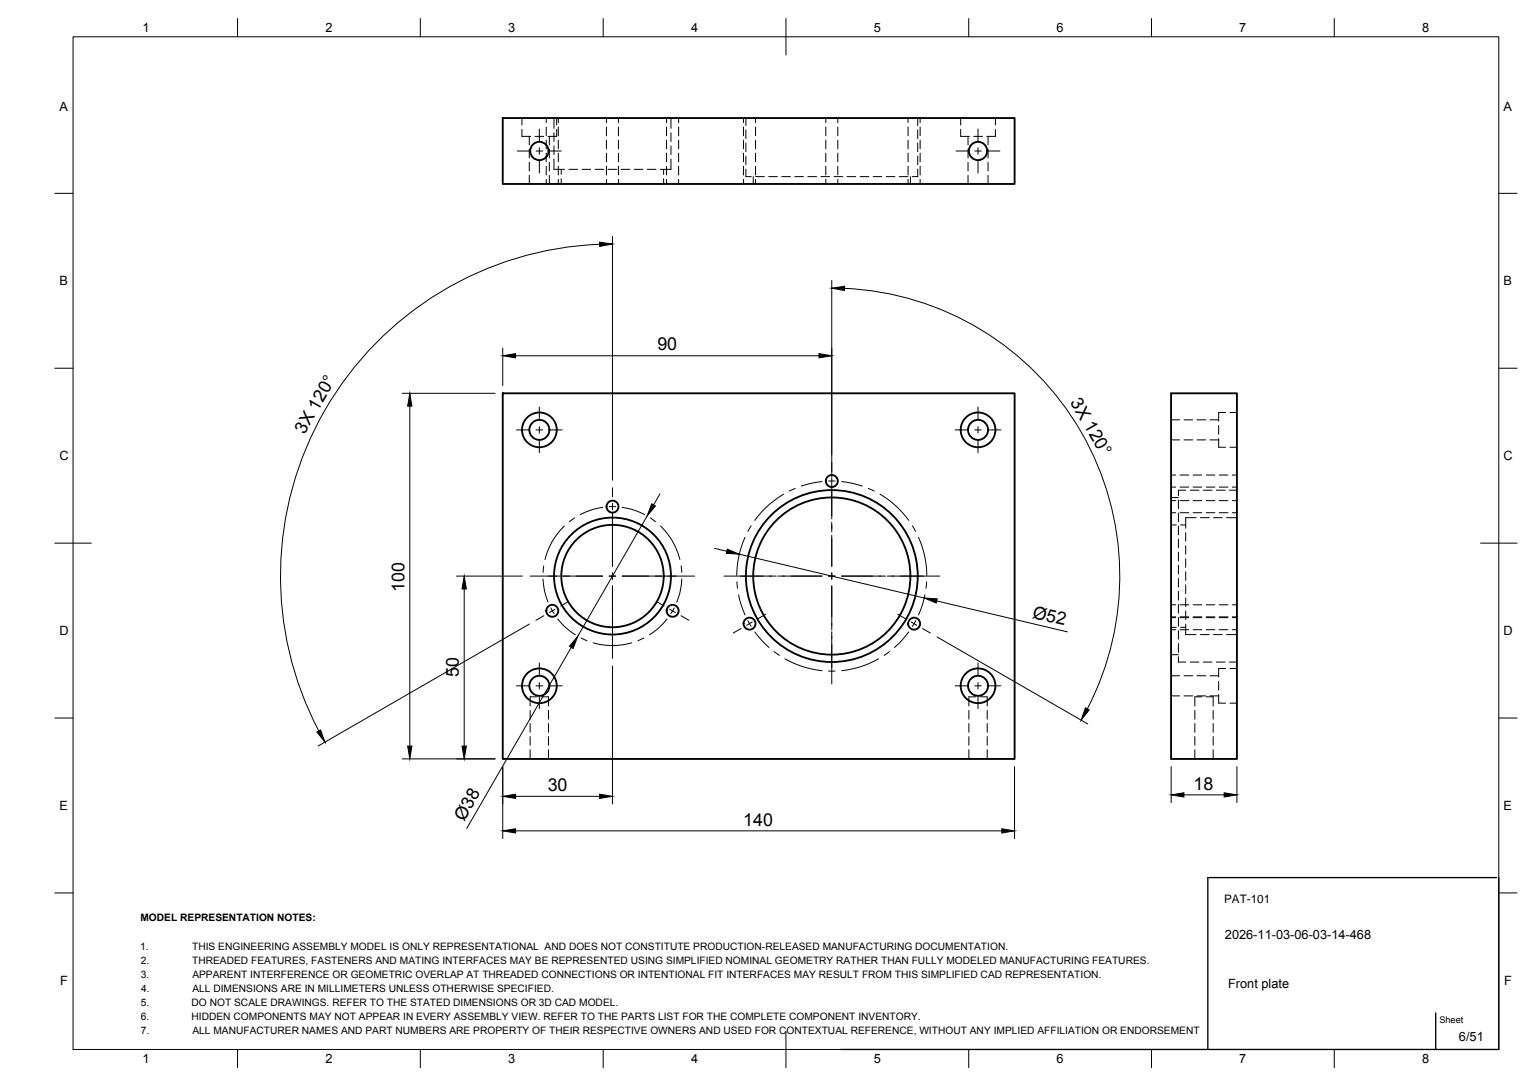
ISO-10303-21;
HEADER;
/* Generated by software containing ST-Developer
 * from STEP Tools, Inc. (www.steptools.com) 
 */

FILE_DESCRIPTION(
/* description */ ('Spur gear reduction stage 2-1 on bearing plates'),
/* implementation_level */ '2;1');

FILE_NAME(
/* name */ 'Front plate.step',
/* time_stamp */ '2026-10-28T03:22:07-07:00',
/* author */ (''),
/* organization */ (''),
/* preprocessor_version */ 'ST-DEVELOPER v20.2',
/* originating_system */ 'Autodesk Translation Framework v15.17.0.0',
/* authorisation */ '');

FILE_SCHEMA (('AUTOMOTIVE_DESIGN { 1 0 10303 214 3 1 1 }'));
ENDSEC;

DATA;
#10=MECHANICAL_DESIGN_GEOMETRIC_PRESENTATION_REPRESENTATION('',(#948),#53909);
#862=SHAPE_REPRESENTATION_RELATIONSHIP('SRR','None',#54089,#905);
#905=ADVANCED_BREP_SHAPE_REPRESENTATION('',(#1006),#53863);
#948=STYLED_ITEM('',(#54411),#1006);
#1006=MANIFOLD_SOLID_BREP('Body1',#11272);
#1068=FACE_BOUND('',#2177,.T.);
#1069=FACE_BOUND('',#2180,.T.);
#1070=FACE_BOUND('',#2183,.T.);
#1071=FACE_BOUND('',#2186,.T.);
#1072=FACE_BOUND('',#2197,.T.);
#1073=FACE_BOUND('',#2201,.T.);
#1074=FACE_BOUND('',#2204,.T.);
#1075=FACE_BOUND('',#2205,.T.);
#1076=FACE_BOUND('',#2206,.T.);
#1077=FACE_BOUND('',#2207,.T.);
#1078=FACE_BOUND('',#2208,.T.);
#1079=FACE_BOUND('',#2209,.T.);
#1080=FACE_BOUND('',#2210,.T.);
#1081=FACE_BOUND('',#2211,.T.);
#1082=FACE_BOUND('',#2212,.T.);
#1083=FACE_BOUND('',#2213,.T.);
#1084=FACE_BOUND('',#2214,.T.);
#1085=FACE_BOUND('',#2215,.T.);
#1086=FACE_BOUND('',#2218,.T.);
#1087=FACE_BOUND('',#2219,.T.);
#1088=FACE_BOUND('',#2220,.T.);
#1089=FACE_BOUND('',#2221,.T.);
#1090=FACE_BOUND('',#2222,.T.);
#1091=FACE_BOUND('',#2223,.T.);
#1092=FACE_BOUND('',#2224,.T.);
#1093=FACE_BOUND('',#2225,.T.);
#1094=FACE_BOUND('',#2226,.T.);
#1095=FACE_BOUND('',#2227,.T.);
#1096=FACE_BOUND('',#2228,.T.);
#1097=FACE_BOUND('',#2229,.T.);
#1098=FACE_BOUND('',#2233,.T.);
#1099=FACE_BOUND('',#2234,.T.);
#1244=PLANE('',#11849);
#1245=PLANE('',#11854);
#1246=PLANE('',#11859);
#1247=PLANE('',#11864);
#1248=PLANE('',#11877);
#1249=PLANE('',#11881);
#1250=PLANE('',#11885);
#1251=PLANE('',#11892);
#1252=PLANE('',#11896);
#1253=PLANE('',#11897);
#1254=PLANE('',#11898);
#1255=PLANE('',#11899);
#1256=PLANE('',#11900);
#1257=PLANE('',#11901);
#1513=FACE_OUTER_BOUND('',#2169,.T.);
#1514=FACE_OUTER_BOUND('',#2170,.T.);
#1515=FACE_OUTER_BOUND('',#2171,.T.);
#1516=FACE_OUTER_BOUND('',#2172,.T.);
#1517=FACE_OUTER_BOUND('',#2173,.T.);
#1518=FACE_OUTER_BOUND('',#2174,.T.);
#1519=FACE_OUTER_BOUND('',#2175,.T.);
#1520=FACE_OUTER_BOUND('',#2176,.T.);
#1521=FACE_OUTER_BOUND('',#2178,.T.);
#1522=FACE_OUTER_BOUND('',#2179,.T.);
#1523=FACE_OUTER_BOUND('',#2181,.T.);
#1524=FACE_OUTER_BOUND('',#2182,.T.);
#1525=FACE_OUTER_BOUND('',#2184,.T.);
#1526=FACE_OUTER_BOUND('',#2185,.T.);
#1527=FACE_OUTER_BOUND('',#2187,.T.);
#1528=FACE_OUTER_BOUND('',#2188,.T.);
#1529=FACE_OUTER_BOUND('',#2189,.T.);
#1530=FACE_OUTER_BOUND('',#2190,.T.);
#1531=FACE_OUTER_BOUND('',#2191,.T.);
#1532=FACE_OUTER_BOUND('',#2192,.T.);
#1533=FACE_OUTER_BOUND('',#2193,.T.);
#1534=FACE_OUTER_BOUND('',#2194,.T.);
#1535=FACE_OUTER_BOUND('',#2195,.T.);
#1536=FACE_OUTER_BOUND('',#2196,.T.);
#1537=FACE_OUTER_BOUND('',#2198,.T.);
#1538=FACE_OUTER_BOUND('',#2199,.T.);
#1539=FACE_OUTER_BOUND('',#2200,.T.);
#1540=FACE_OUTER_BOUND('',#2202,.T.);
#1541=FACE_OUTER_BOUND('',#2203,.T.);
#1542=FACE_OUTER_BOUND('',#2216,.T.);
#1543=FACE_OUTER_BOUND('',#2217,.T.);
#1544=FACE_OUTER_BOUND('',#2230,.T.);
#1545=FACE_OUTER_BOUND('',#2231,.T.);
#1546=FACE_OUTER_BOUND('',#2232,.T.);
#2169=EDGE_LOOP('',(#7400,#7401,#7402,#7403));
#2170=EDGE_LOOP('',(#7404,#7405,#7406,#7407));
#2171=EDGE_LOOP('',(#7408,#7409,#7410,#7411));
#2172=EDGE_LOOP('',(#7412,#7413,#7414,#7415));
#2173=EDGE_LOOP('',(#7416,#7417,#7418,#7419));
#2174=EDGE_LOOP('',(#7420,#7421,#7422,#7423));
#2175=EDGE_LOOP('',(#7424,#7425,#7426,#7427));
#2176=EDGE_LOOP('',(#7428));
#2177=EDGE_LOOP('',(#7429));
#2178=EDGE_LOOP('',(#7430,#7431,#7432,#7433));
#2179=EDGE_LOOP('',(#7434));
#2180=EDGE_LOOP('',(#7435));
#2181=EDGE_LOOP('',(#7436,#7437,#7438,#7439));
#2182=EDGE_LOOP('',(#7440));
#2183=EDGE_LOOP('',(#7441));
#2184=EDGE_LOOP('',(#7442,#7443,#7444,#7445));
#2185=EDGE_LOOP('',(#7446));
#2186=EDGE_LOOP('',(#7447));
#2187=EDGE_LOOP('',(#7448,#7449,#7450,#7451));
#2188=EDGE_LOOP('',(#7452,#7453,#7454,#7455));
#2189=EDGE_LOOP('',(#7456,#7457,#7458,#7459));
#2190=EDGE_LOOP('',(#7460,#7461,#7462,#7463));
#2191=EDGE_LOOP('',(#7464,#7465,#7466,#7467));
#2192=EDGE_LOOP('',(#7468));
#2193=EDGE_LOOP('',(#7469,#7470,#7471,#7472));
#2194=EDGE_LOOP('',(#7473));
#2195=EDGE_LOOP('',(#7474,#7475,#7476,#7477));
#2196=EDGE_LOOP('',(#7478));
#2197=EDGE_LOOP('',(#7479));
#2198=EDGE_LOOP('',(#7480,#7481,#7482,#7483));
#2199=EDGE_LOOP('',(#7484,#7485,#7486,#7487));
#2200=EDGE_LOOP('',(#7488));
#2201=EDGE_LOOP('',(#7489));
#2202=EDGE_LOOP('',(#7490,#7491,#7492,#7493));
#2203=EDGE_LOOP('',(#7494,#7495,#7496,#7497));
#2204=EDGE_LOOP('',(#7498));
#2205=EDGE_LOOP('',(#7499));
#2206=EDGE_LOOP('',(#7500));
#2207=EDGE_LOOP('',(#7501));
#2208=EDGE_LOOP('',(#7502));
#2209=EDGE_LOOP('',(#7503));
#2210=EDGE_LOOP('',(#7504));
#2211=EDGE_LOOP('',(#7505));
#2212=EDGE_LOOP('',(#7506));
#2213=EDGE_LOOP('',(#7507));
#2214=EDGE_LOOP('',(#7508));
#2215=EDGE_LOOP('',(#7509));
#2216=EDGE_LOOP('',(#7510,#7511,#7512,#7513));
#2217=EDGE_LOOP('',(#7514,#7515,#7516,#7517));
#2218=EDGE_LOOP('',(#7518));
#2219=EDGE_LOOP('',(#7519));
#2220=EDGE_LOOP('',(#7520));
#2221=EDGE_LOOP('',(#7521));
#2222=EDGE_LOOP('',(#7522));
#2223=EDGE_LOOP('',(#7523));
#2224=EDGE_LOOP('',(#7524));
#2225=EDGE_LOOP('',(#7525));
#2226=EDGE_LOOP('',(#7526));
#2227=EDGE_LOOP('',(#7527));
#2228=EDGE_LOOP('',(#7528));
#2229=EDGE_LOOP('',(#7529));
#2230=EDGE_LOOP('',(#7530,#7531,#7532,#7533));
#2231=EDGE_LOOP('',(#7534,#7535,#7536,#7537));
#2232=EDGE_LOOP('',(#7538,#7539,#7540,#7541));
#2233=EDGE_LOOP('',(#7542));
#2234=EDGE_LOOP('',(#7543));
#2993=LINE('',#16033,#3634);
#2994=LINE('',#16039,#3635);
#2995=LINE('',#16045,#3636);
#2996=LINE('',#16051,#3637);
#2997=LINE('',#16057,#3638);
#2998=LINE('',#16063,#3639);
#2999=LINE('',#16069,#3640);
#3000=LINE('',#16078,#3641);
#3001=LINE('',#16087,#3642);
#3002=LINE('',#16096,#3643);
#3003=LINE('',#16103,#3644);
#3004=LINE('',#16107,#3645);
#3005=LINE('',#16111,#3646);
#3006=LINE('',#16115,#3647);
#3007=LINE('',#16121,#3648);
#3008=LINE('',#16128,#3649);
#3009=LINE('',#16135,#3650);
#3010=LINE('',#16142,#3651);
#3011=LINE('',#16148,#3652);
#3012=LINE('',#16155,#3653);
#3013=LINE('',#16160,#3654);
#3014=LINE('',#16162,#3655);
#3015=LINE('',#16164,#3656);
#3016=LINE('',#16165,#3657);
#3017=LINE('',#16168,#3658);
#3018=LINE('',#16170,#3659);
#3019=LINE('',#16171,#3660);
#3020=LINE('',#16174,#3661);
#3021=LINE('',#16176,#3662);
#3022=LINE('',#16177,#3663);
#3023=LINE('',#16179,#3664);
#3024=LINE('',#16180,#3665);
#3634=VECTOR('',#13046,0.165);
#3635=VECTOR('',#13053,0.165);
#3636=VECTOR('',#13060,0.164999999999999);
#3637=VECTOR('',#13067,0.165);
#3638=VECTOR('',#13074,0.165);
#3639=VECTOR('',#13081,0.165);
#3640=VECTOR('',#13088,0.475);
#3641=VECTOR('',#13099,0.475);
#3642=VECTOR('',#13110,0.475);
#3643=VECTOR('',#13121,0.475);
#3644=VECTOR('',#13130,0.275);
#3645=VECTOR('',#13135,0.275);
#3646=VECTOR('',#13140,0.275);
#3647=VECTOR('',#13145,0.275);
#3648=VECTOR('',#13152,0.25);
#3649=VECTOR('',#13161,0.25);
#3650=VECTOR('',#13170,2.35);
#3651=VECTOR('',#13179,2.15);
#3652=VECTOR('',#13186,1.6);
#3653=VECTOR('',#13195,1.4);
#3654=VECTOR('',#13200,1.);
#3655=VECTOR('',#13201,1.);
#3656=VECTOR('',#13202,1.);
#3657=VECTOR('',#13203,1.);
#3658=VECTOR('',#13206,1.);
#3659=VECTOR('',#13207,1.);
#3660=VECTOR('',#13208,1.);
#3661=VECTOR('',#13211,1.);
#3662=VECTOR('',#13212,1.);
#3663=VECTOR('',#13213,1.);
#3664=VECTOR('',#13216,1.);
#3665=VECTOR('',#13217,1.);
#4267=CIRCLE('',#11829,0.165);
#4268=CIRCLE('',#11830,0.165);
#4269=CIRCLE('',#11832,0.165);
#4270=CIRCLE('',#11833,0.165);
#4271=CIRCLE('',#11835,0.164999999999999);
#4272=CIRCLE('',#11836,0.164999999999999);
#4273=CIRCLE('',#11838,0.165);
#4274=CIRCLE('',#11839,0.165);
#4275=CIRCLE('',#11841,0.165);
#4276=CIRCLE('',#11842,0.165);
#4277=CIRCLE('',#11844,0.165);
#4278=CIRCLE('',#11845,0.165);
#4279=CIRCLE('',#11847,0.475);
#4280=CIRCLE('',#11848,0.475);
#4281=CIRCLE('',#11850,0.275);
#4282=CIRCLE('',#11852,0.475);
#4283=CIRCLE('',#11853,0.475);
#4284=CIRCLE('',#11855,0.275);
#4285=CIRCLE('',#11857,0.475);
#4286=CIRCLE('',#11858,0.475);
#4287=CIRCLE('',#11860,0.275);
#4288=CIRCLE('',#11862,0.475);
#4289=CIRCLE('',#11863,0.475);
#4290=CIRCLE('',#11865,0.275);
#4291=CIRCLE('',#11867,0.275);
#4292=CIRCLE('',#11869,0.275);
#4293=CIRCLE('',#11871,0.275);
#4294=CIRCLE('',#11873,0.275);
#4295=CIRCLE('',#11875,0.25);
#4296=CIRCLE('',#11876,0.25);
#4297=CIRCLE('',#11879,0.25);
#4298=CIRCLE('',#11880,0.25);
#4299=CIRCLE('',#11883,2.35);
#4300=CIRCLE('',#11884,2.35);
#4301=CIRCLE('',#11886,2.15);
#4302=CIRCLE('',#11888,2.15);
#4303=CIRCLE('',#11890,1.6);
#4304=CIRCLE('',#11891,1.6);
#4305=CIRCLE('',#11893,1.4);
#4306=CIRCLE('',#11895,1.4);
#4800=VERTEX_POINT('',#16030);
#4801=VERTEX_POINT('',#16032);
#4802=VERTEX_POINT('',#16036);
#4803=VERTEX_POINT('',#16038);
#4804=VERTEX_POINT('',#16042);
#4805=VERTEX_POINT('',#16044);
#4806=VERTEX_POINT('',#16048);
#4807=VERTEX_POINT('',#16050);
#4808=VERTEX_POINT('',#16054);
#4809=VERTEX_POINT('',#16056);
#4810=VERTEX_POINT('',#16060);
#4811=VERTEX_POINT('',#16062);
#4812=VERTEX_POINT('',#16066);
#4813=VERTEX_POINT('',#16068);
#4814=VERTEX_POINT('',#16072);
#4815=VERTEX_POINT('',#16075);
#4816=VERTEX_POINT('',#16077);
#4817=VERTEX_POINT('',#16081);
#4818=VERTEX_POINT('',#16084);
#4819=VERTEX_POINT('',#16086);
#4820=VERTEX_POINT('',#16090);
#4821=VERTEX_POINT('',#16093);
#4822=VERTEX_POINT('',#16095);
#4823=VERTEX_POINT('',#16099);
#4824=VERTEX_POINT('',#16102);
#4825=VERTEX_POINT('',#16106);
#4826=VERTEX_POINT('',#16110);
#4827=VERTEX_POINT('',#16114);
#4828=VERTEX_POINT('',#16118);
#4829=VERTEX_POINT('',#16120);
#4830=VERTEX_POINT('',#16125);
#4831=VERTEX_POINT('',#16127);
#4832=VERTEX_POINT('',#16132);
#4833=VERTEX_POINT('',#16134);
#4834=VERTEX_POINT('',#16138);
#4835=VERTEX_POINT('',#16141);
#4836=VERTEX_POINT('',#16145);
#4837=VERTEX_POINT('',#16147);
#4838=VERTEX_POINT('',#16151);
#4839=VERTEX_POINT('',#16154);
#4840=VERTEX_POINT('',#16158);
#4841=VERTEX_POINT('',#16159);
#4842=VERTEX_POINT('',#16161);
#4843=VERTEX_POINT('',#16163);
#4844=VERTEX_POINT('',#16167);
#4845=VERTEX_POINT('',#16169);
#4846=VERTEX_POINT('',#16173);
#4847=VERTEX_POINT('',#16175);
#5842=EDGE_CURVE('',#4800,#4800,#4267,.T.);
#5843=EDGE_CURVE('',#4800,#4801,#2993,.T.);
#5844=EDGE_CURVE('',#4801,#4801,#4268,.T.);
#5845=EDGE_CURVE('',#4802,#4802,#4269,.T.);
#5846=EDGE_CURVE('',#4802,#4803,#2994,.T.);
#5847=EDGE_CURVE('',#4803,#4803,#4270,.T.);
#5848=EDGE_CURVE('',#4804,#4804,#4271,.T.);
#5849=EDGE_CURVE('',#4804,#4805,#2995,.T.);
#5850=EDGE_CURVE('',#4805,#4805,#4272,.T.);
#5851=EDGE_CURVE('',#4806,#4806,#4273,.T.);
#5852=EDGE_CURVE('',#4806,#4807,#2996,.T.);
#5853=EDGE_CURVE('',#4807,#4807,#4274,.T.);
#5854=EDGE_CURVE('',#4808,#4808,#4275,.T.);
#5855=EDGE_CURVE('',#4808,#4809,#2997,.T.);
#5856=EDGE_CURVE('',#4809,#4809,#4276,.T.);
#5857=EDGE_CURVE('',#4810,#4810,#4277,.T.);
#5858=EDGE_CURVE('',#4810,#4811,#2998,.T.);
#5859=EDGE_CURVE('',#4811,#4811,#4278,.T.);
#5860=EDGE_CURVE('',#4812,#4812,#4279,.T.);
#5861=EDGE_CURVE('',#4812,#4813,#2999,.T.);
#5862=EDGE_CURVE('',#4813,#4813,#4280,.T.);
#5863=EDGE_CURVE('',#4814,#4814,#4281,.T.);
#5864=EDGE_CURVE('',#4815,#4815,#4282,.T.);
#5865=EDGE_CURVE('',#4815,#4816,#3000,.T.);
#5866=EDGE_CURVE('',#4816,#4816,#4283,.T.);
#5867=EDGE_CURVE('',#4817,#4817,#4284,.T.);
#5868=EDGE_CURVE('',#4818,#4818,#4285,.T.);
#5869=EDGE_CURVE('',#4818,#4819,#3001,.T.);
#5870=EDGE_CURVE('',#4819,#4819,#4286,.T.);
#5871=EDGE_CURVE('',#4820,#4820,#4287,.T.);
#5872=EDGE_CURVE('',#4821,#4821,#4288,.T.);
#5873=EDGE_CURVE('',#4821,#4822,#3002,.T.);
#5874=EDGE_CURVE('',#4822,#4822,#4289,.T.);
#5875=EDGE_CURVE('',#4823,#4823,#4290,.T.);
#5876=EDGE_CURVE('',#4814,#4824,#3003,.T.);
#5877=EDGE_CURVE('',#4824,#4824,#4291,.T.);
#5878=EDGE_CURVE('',#4817,#4825,#3004,.T.);
#5879=EDGE_CURVE('',#4825,#4825,#4292,.T.);
#5880=EDGE_CURVE('',#4820,#4826,#3005,.T.);
#5881=EDGE_CURVE('',#4826,#4826,#4293,.T.);
#5882=EDGE_CURVE('',#4823,#4827,#3006,.T.);
#5883=EDGE_CURVE('',#4827,#4827,#4294,.T.);
#5884=EDGE_CURVE('',#4828,#4828,#4295,.T.);
#5885=EDGE_CURVE('',#4828,#4829,#3007,.T.);
#5886=EDGE_CURVE('',#4829,#4829,#4296,.T.);
#5887=EDGE_CURVE('',#4830,#4830,#4297,.T.);
#5888=EDGE_CURVE('',#4830,#4831,#3008,.T.);
#5889=EDGE_CURVE('',#4831,#4831,#4298,.T.);
#5890=EDGE_CURVE('',#4832,#4832,#4299,.T.);
#5891=EDGE_CURVE('',#4832,#4833,#3009,.T.);
#5892=EDGE_CURVE('',#4833,#4833,#4300,.T.);
#5893=EDGE_CURVE('',#4834,#4834,#4301,.T.);
#5894=EDGE_CURVE('',#4834,#4835,#3010,.T.);
#5895=EDGE_CURVE('',#4835,#4835,#4302,.T.);
#5896=EDGE_CURVE('',#4836,#4836,#4303,.T.);
#5897=EDGE_CURVE('',#4836,#4837,#3011,.T.);
#5898=EDGE_CURVE('',#4837,#4837,#4304,.T.);
#5899=EDGE_CURVE('',#4838,#4838,#4305,.T.);
#5900=EDGE_CURVE('',#4838,#4839,#3012,.T.);
#5901=EDGE_CURVE('',#4839,#4839,#4306,.T.);
#5902=EDGE_CURVE('',#4840,#4841,#3013,.T.);
#5903=EDGE_CURVE('',#4841,#4842,#3014,.T.);
#5904=EDGE_CURVE('',#4843,#4842,#3015,.T.);
#5905=EDGE_CURVE('',#4840,#4843,#3016,.T.);
#5906=EDGE_CURVE('',#4844,#4840,#3017,.T.);
#5907=EDGE_CURVE('',#4845,#4843,#3018,.T.);
#5908=EDGE_CURVE('',#4844,#4845,#3019,.T.);
#5909=EDGE_CURVE('',#4846,#4844,#3020,.T.);
#5910=EDGE_CURVE('',#4847,#4845,#3021,.T.);
#5911=EDGE_CURVE('',#4846,#4847,#3022,.T.);
#5912=EDGE_CURVE('',#4841,#4846,#3023,.T.);
#5913=EDGE_CURVE('',#4842,#4847,#3024,.T.);
#7400=ORIENTED_EDGE('',*,*,#5842,.F.);
#7401=ORIENTED_EDGE('',*,*,#5843,.T.);
#7402=ORIENTED_EDGE('',*,*,#5844,.F.);
#7403=ORIENTED_EDGE('',*,*,#5843,.F.);
#7404=ORIENTED_EDGE('',*,*,#5845,.F.);
#7405=ORIENTED_EDGE('',*,*,#5846,.T.);
#7406=ORIENTED_EDGE('',*,*,#5847,.F.);
#7407=ORIENTED_EDGE('',*,*,#5846,.F.);
#7408=ORIENTED_EDGE('',*,*,#5848,.F.);
#7409=ORIENTED_EDGE('',*,*,#5849,.T.);
#7410=ORIENTED_EDGE('',*,*,#5850,.F.);
#7411=ORIENTED_EDGE('',*,*,#5849,.F.);
#7412=ORIENTED_EDGE('',*,*,#5851,.F.);
#7413=ORIENTED_EDGE('',*,*,#5852,.T.);
#7414=ORIENTED_EDGE('',*,*,#5853,.F.);
#7415=ORIENTED_EDGE('',*,*,#5852,.F.);
#7416=ORIENTED_EDGE('',*,*,#5854,.F.);
#7417=ORIENTED_EDGE('',*,*,#5855,.T.);
#7418=ORIENTED_EDGE('',*,*,#5856,.F.);
#7419=ORIENTED_EDGE('',*,*,#5855,.F.);
#7420=ORIENTED_EDGE('',*,*,#5857,.F.);
#7421=ORIENTED_EDGE('',*,*,#5858,.T.);
#7422=ORIENTED_EDGE('',*,*,#5859,.F.);
#7423=ORIENTED_EDGE('',*,*,#5858,.F.);
#7424=ORIENTED_EDGE('',*,*,#5860,.F.);
#7425=ORIENTED_EDGE('',*,*,#5861,.T.);
#7426=ORIENTED_EDGE('',*,*,#5862,.T.);
#7427=ORIENTED_EDGE('',*,*,#5861,.F.);
#7428=ORIENTED_EDGE('',*,*,#5862,.F.);
#7429=ORIENTED_EDGE('',*,*,#5863,.F.);
#7430=ORIENTED_EDGE('',*,*,#5864,.F.);
#7431=ORIENTED_EDGE('',*,*,#5865,.T.);
#7432=ORIENTED_EDGE('',*,*,#5866,.T.);
#7433=ORIENTED_EDGE('',*,*,#5865,.F.);
#7434=ORIENTED_EDGE('',*,*,#5866,.F.);
#7435=ORIENTED_EDGE('',*,*,#5867,.F.);
#7436=ORIENTED_EDGE('',*,*,#5868,.F.);
#7437=ORIENTED_EDGE('',*,*,#5869,.T.);
#7438=ORIENTED_EDGE('',*,*,#5870,.T.);
#7439=ORIENTED_EDGE('',*,*,#5869,.F.);
#7440=ORIENTED_EDGE('',*,*,#5870,.F.);
#7441=ORIENTED_EDGE('',*,*,#5871,.F.);
#7442=ORIENTED_EDGE('',*,*,#5872,.F.);
#7443=ORIENTED_EDGE('',*,*,#5873,.T.);
#7444=ORIENTED_EDGE('',*,*,#5874,.T.);
#7445=ORIENTED_EDGE('',*,*,#5873,.F.);
#7446=ORIENTED_EDGE('',*,*,#5874,.F.);
#7447=ORIENTED_EDGE('',*,*,#5875,.F.);
#7448=ORIENTED_EDGE('',*,*,#5863,.T.);
#7449=ORIENTED_EDGE('',*,*,#5876,.T.);
#7450=ORIENTED_EDGE('',*,*,#5877,.F.);
#7451=ORIENTED_EDGE('',*,*,#5876,.F.);
#7452=ORIENTED_EDGE('',*,*,#5867,.T.);
#7453=ORIENTED_EDGE('',*,*,#5878,.T.);
#7454=ORIENTED_EDGE('',*,*,#5879,.F.);
#7455=ORIENTED_EDGE('',*,*,#5878,.F.);
#7456=ORIENTED_EDGE('',*,*,#5871,.T.);
#7457=ORIENTED_EDGE('',*,*,#5880,.T.);
#7458=ORIENTED_EDGE('',*,*,#5881,.F.);
#7459=ORIENTED_EDGE('',*,*,#5880,.F.);
#7460=ORIENTED_EDGE('',*,*,#5875,.T.);
#7461=ORIENTED_EDGE('',*,*,#5882,.T.);
#7462=ORIENTED_EDGE('',*,*,#5883,.F.);
#7463=ORIENTED_EDGE('',*,*,#5882,.F.);
#7464=ORIENTED_EDGE('',*,*,#5884,.F.);
#7465=ORIENTED_EDGE('',*,*,#5885,.T.);
#7466=ORIENTED_EDGE('',*,*,#5886,.T.);
#7467=ORIENTED_EDGE('',*,*,#5885,.F.);
#7468=ORIENTED_EDGE('',*,*,#5886,.F.);
#7469=ORIENTED_EDGE('',*,*,#5887,.F.);
#7470=ORIENTED_EDGE('',*,*,#5888,.T.);
#7471=ORIENTED_EDGE('',*,*,#5889,.T.);
#7472=ORIENTED_EDGE('',*,*,#5888,.F.);
#7473=ORIENTED_EDGE('',*,*,#5889,.F.);
#7474=ORIENTED_EDGE('',*,*,#5890,.F.);
#7475=ORIENTED_EDGE('',*,*,#5891,.T.);
#7476=ORIENTED_EDGE('',*,*,#5892,.T.);
#7477=ORIENTED_EDGE('',*,*,#5891,.F.);
#7478=ORIENTED_EDGE('',*,*,#5892,.F.);
#7479=ORIENTED_EDGE('',*,*,#5893,.F.);
#7480=ORIENTED_EDGE('',*,*,#5893,.T.);
#7481=ORIENTED_EDGE('',*,*,#5894,.T.);
#7482=ORIENTED_EDGE('',*,*,#5895,.F.);
#7483=ORIENTED_EDGE('',*,*,#5894,.F.);
#7484=ORIENTED_EDGE('',*,*,#5896,.F.);
#7485=ORIENTED_EDGE('',*,*,#5897,.T.);
#7486=ORIENTED_EDGE('',*,*,#5898,.T.);
#7487=ORIENTED_EDGE('',*,*,#5897,.F.);
#7488=ORIENTED_EDGE('',*,*,#5898,.F.);
#7489=ORIENTED_EDGE('',*,*,#5899,.F.);
#7490=ORIENTED_EDGE('',*,*,#5899,.T.);
#7491=ORIENTED_EDGE('',*,*,#5900,.T.);
#7492=ORIENTED_EDGE('',*,*,#5901,.F.);
#7493=ORIENTED_EDGE('',*,*,#5900,.F.);
#7494=ORIENTED_EDGE('',*,*,#5902,.T.);
#7495=ORIENTED_EDGE('',*,*,#5903,.T.);
#7496=ORIENTED_EDGE('',*,*,#5904,.F.);
#7497=ORIENTED_EDGE('',*,*,#5905,.F.);
#7498=ORIENTED_EDGE('',*,*,#5853,.T.);
#7499=ORIENTED_EDGE('',*,*,#5856,.T.);
#7500=ORIENTED_EDGE('',*,*,#5859,.T.);
#7501=ORIENTED_EDGE('',*,*,#5901,.T.);
#7502=ORIENTED_EDGE('',*,*,#5895,.T.);
#7503=ORIENTED_EDGE('',*,*,#5883,.T.);
#7504=ORIENTED_EDGE('',*,*,#5881,.T.);
#7505=ORIENTED_EDGE('',*,*,#5879,.T.);
#7506=ORIENTED_EDGE('',*,*,#5877,.T.);
#7507=ORIENTED_EDGE('',*,*,#5850,.T.);
#7508=ORIENTED_EDGE('',*,*,#5847,.T.);
#7509=ORIENTED_EDGE('',*,*,#5844,.T.);
#7510=ORIENTED_EDGE('',*,*,#5906,.T.);
#7511=ORIENTED_EDGE('',*,*,#5905,.T.);
#7512=ORIENTED_EDGE('',*,*,#5907,.F.);
#7513=ORIENTED_EDGE('',*,*,#5908,.F.);
#7514=ORIENTED_EDGE('',*,*,#5909,.T.);
#7515=ORIENTED_EDGE('',*,*,#5908,.T.);
#7516=ORIENTED_EDGE('',*,*,#5910,.F.);
#7517=ORIENTED_EDGE('',*,*,#5911,.F.);
#7518=ORIENTED_EDGE('',*,*,#5851,.T.);
#7519=ORIENTED_EDGE('',*,*,#5854,.T.);
#7520=ORIENTED_EDGE('',*,*,#5857,.T.);
#7521=ORIENTED_EDGE('',*,*,#5890,.T.);
#7522=ORIENTED_EDGE('',*,*,#5896,.T.);
#7523=ORIENTED_EDGE('',*,*,#5872,.T.);
#7524=ORIENTED_EDGE('',*,*,#5868,.T.);
#7525=ORIENTED_EDGE('',*,*,#5864,.T.);
#7526=ORIENTED_EDGE('',*,*,#5860,.T.);
#7527=ORIENTED_EDGE('',*,*,#5848,.T.);
#7528=ORIENTED_EDGE('',*,*,#5845,.T.);
#7529=ORIENTED_EDGE('',*,*,#5842,.T.);
#7530=ORIENTED_EDGE('',*,*,#5912,.T.);
#7531=ORIENTED_EDGE('',*,*,#5911,.T.);
#7532=ORIENTED_EDGE('',*,*,#5913,.F.);
#7533=ORIENTED_EDGE('',*,*,#5903,.F.);
#7534=ORIENTED_EDGE('',*,*,#5913,.T.);
#7535=ORIENTED_EDGE('',*,*,#5910,.T.);
#7536=ORIENTED_EDGE('',*,*,#5907,.T.);
#7537=ORIENTED_EDGE('',*,*,#5904,.T.);
#7538=ORIENTED_EDGE('',*,*,#5912,.F.);
#7539=ORIENTED_EDGE('',*,*,#5902,.F.);
#7540=ORIENTED_EDGE('',*,*,#5906,.F.);
#7541=ORIENTED_EDGE('',*,*,#5909,.F.);
#7542=ORIENTED_EDGE('',*,*,#5884,.T.);
#7543=ORIENTED_EDGE('',*,*,#5887,.T.);
#10424=CYLINDRICAL_SURFACE('',#11828,0.165);
#10425=CYLINDRICAL_SURFACE('',#11831,0.165);
#10426=CYLINDRICAL_SURFACE('',#11834,0.164999999999999);
#10427=CYLINDRICAL_SURFACE('',#11837,0.165);
#10428=CYLINDRICAL_SURFACE('',#11840,0.165);
#10429=CYLINDRICAL_SURFACE('',#11843,0.165);
#10430=CYLINDRICAL_SURFACE('',#11846,0.475);
#10431=CYLINDRICAL_SURFACE('',#11851,0.475);
#10432=CYLINDRICAL_SURFACE('',#11856,0.475);
#10433=CYLINDRICAL_SURFACE('',#11861,0.475);
#10434=CYLINDRICAL_SURFACE('',#11866,0.275);
#10435=CYLINDRICAL_SURFACE('',#11868,0.275);
#10436=CYLINDRICAL_SURFACE('',#11870,0.275);
#10437=CYLINDRICAL_SURFACE('',#11872,0.275);
#10438=CYLINDRICAL_SURFACE('',#11874,0.25);
#10439=CYLINDRICAL_SURFACE('',#11878,0.25);
#10440=CYLINDRICAL_SURFACE('',#11882,2.35);
#10441=CYLINDRICAL_SURFACE('',#11887,2.15);
#10442=CYLINDRICAL_SURFACE('',#11889,1.6);
#10443=CYLINDRICAL_SURFACE('',#11894,1.4);
#10633=ADVANCED_FACE('',(#1513),#10424,.F.);
#10634=ADVANCED_FACE('',(#1514),#10425,.F.);
#10635=ADVANCED_FACE('',(#1515),#10426,.F.);
#10636=ADVANCED_FACE('',(#1516),#10427,.F.);
#10637=ADVANCED_FACE('',(#1517),#10428,.F.);
#10638=ADVANCED_FACE('',(#1518),#10429,.F.);
#10639=ADVANCED_FACE('',(#1519),#10430,.F.);
#10640=ADVANCED_FACE('',(#1520,#1068),#1244,.F.);
#10641=ADVANCED_FACE('',(#1521),#10431,.F.);
#10642=ADVANCED_FACE('',(#1522,#1069),#1245,.F.);
#10643=ADVANCED_FACE('',(#1523),#10432,.F.);
#10644=ADVANCED_FACE('',(#1524,#1070),#1246,.F.);
#10645=ADVANCED_FACE('',(#1525),#10433,.F.);
#10646=ADVANCED_FACE('',(#1526,#1071),#1247,.F.);
#10647=ADVANCED_FACE('',(#1527),#10434,.F.);
#10648=ADVANCED_FACE('',(#1528),#10435,.F.);
#10649=ADVANCED_FACE('',(#1529),#10436,.F.);
#10650=ADVANCED_FACE('',(#1530),#10437,.F.);
#10651=ADVANCED_FACE('',(#1531),#10438,.F.);
#10652=ADVANCED_FACE('',(#1532),#1248,.F.);
#10653=ADVANCED_FACE('',(#1533),#10439,.F.);
#10654=ADVANCED_FACE('',(#1534),#1249,.F.);
#10655=ADVANCED_FACE('',(#1535),#10440,.F.);
#10656=ADVANCED_FACE('',(#1536,#1072),#1250,.F.);
#10657=ADVANCED_FACE('',(#1537),#10441,.F.);
#10658=ADVANCED_FACE('',(#1538),#10442,.F.);
#10659=ADVANCED_FACE('',(#1539,#1073),#1251,.F.);
#10660=ADVANCED_FACE('',(#1540),#10443,.F.);
#10661=ADVANCED_FACE('',(#1541,#1074,#1075,#1076,#1077,#1078,#1079,#1080,
#1081,#1082,#1083,#1084,#1085),#1252,.T.);
#10662=ADVANCED_FACE('',(#1542),#1253,.T.);
#10663=ADVANCED_FACE('',(#1543,#1086,#1087,#1088,#1089,#1090,#1091,#1092,
#1093,#1094,#1095,#1096,#1097),#1254,.T.);
#10664=ADVANCED_FACE('',(#1544),#1255,.T.);
#10665=ADVANCED_FACE('',(#1545),#1256,.T.);
#10666=ADVANCED_FACE('',(#1546,#1098,#1099),#1257,.F.);
#11272=CLOSED_SHELL('',(#10633,#10634,#10635,#10636,#10637,#10638,#10639,
#10640,#10641,#10642,#10643,#10644,#10645,#10646,#10647,#10648,#10649,#10650,
#10651,#10652,#10653,#10654,#10655,#10656,#10657,#10658,#10659,#10660,#10661,
#10662,#10663,#10664,#10665,#10666));
#11827=AXIS2_PLACEMENT_3D('',#16028,#13040,#13041);
#11828=AXIS2_PLACEMENT_3D('',#16029,#13042,#13043);
#11829=AXIS2_PLACEMENT_3D('',#16031,#13044,#13045);
#11830=AXIS2_PLACEMENT_3D('',#16034,#13047,#13048);
#11831=AXIS2_PLACEMENT_3D('',#16035,#13049,#13050);
#11832=AXIS2_PLACEMENT_3D('',#16037,#13051,#13052);
#11833=AXIS2_PLACEMENT_3D('',#16040,#13054,#13055);
#11834=AXIS2_PLACEMENT_3D('',#16041,#13056,#13057);
#11835=AXIS2_PLACEMENT_3D('',#16043,#13058,#13059);
#11836=AXIS2_PLACEMENT_3D('',#16046,#13061,#13062);
#11837=AXIS2_PLACEMENT_3D('',#16047,#13063,#13064);
#11838=AXIS2_PLACEMENT_3D('',#16049,#13065,#13066);
#11839=AXIS2_PLACEMENT_3D('',#16052,#13068,#13069);
#11840=AXIS2_PLACEMENT_3D('',#16053,#13070,#13071);
#11841=AXIS2_PLACEMENT_3D('',#16055,#13072,#13073);
#11842=AXIS2_PLACEMENT_3D('',#16058,#13075,#13076);
#11843=AXIS2_PLACEMENT_3D('',#16059,#13077,#13078);
#11844=AXIS2_PLACEMENT_3D('',#16061,#13079,#13080);
#11845=AXIS2_PLACEMENT_3D('',#16064,#13082,#13083);
#11846=AXIS2_PLACEMENT_3D('',#16065,#13084,#13085);
#11847=AXIS2_PLACEMENT_3D('',#16067,#13086,#13087);
#11848=AXIS2_PLACEMENT_3D('',#16070,#13089,#13090);
#11849=AXIS2_PLACEMENT_3D('',#16071,#13091,#13092);
#11850=AXIS2_PLACEMENT_3D('',#16073,#13093,#13094);
#11851=AXIS2_PLACEMENT_3D('',#16074,#13095,#13096);
#11852=AXIS2_PLACEMENT_3D('',#16076,#13097,#13098);
#11853=AXIS2_PLACEMENT_3D('',#16079,#13100,#13101);
#11854=AXIS2_PLACEMENT_3D('',#16080,#13102,#13103);
#11855=AXIS2_PLACEMENT_3D('',#16082,#13104,#13105);
#11856=AXIS2_PLACEMENT_3D('',#16083,#13106,#13107);
#11857=AXIS2_PLACEMENT_3D('',#16085,#13108,#13109);
#11858=AXIS2_PLACEMENT_3D('',#16088,#13111,#13112);
#11859=AXIS2_PLACEMENT_3D('',#16089,#13113,#13114);
#11860=AXIS2_PLACEMENT_3D('',#16091,#13115,#13116);
#11861=AXIS2_PLACEMENT_3D('',#16092,#13117,#13118);
#11862=AXIS2_PLACEMENT_3D('',#16094,#13119,#13120);
#11863=AXIS2_PLACEMENT_3D('',#16097,#13122,#13123);
#11864=AXIS2_PLACEMENT_3D('',#16098,#13124,#13125);
#11865=AXIS2_PLACEMENT_3D('',#16100,#13126,#13127);
#11866=AXIS2_PLACEMENT_3D('',#16101,#13128,#13129);
#11867=AXIS2_PLACEMENT_3D('',#16104,#13131,#13132);
#11868=AXIS2_PLACEMENT_3D('',#16105,#13133,#13134);
#11869=AXIS2_PLACEMENT_3D('',#16108,#13136,#13137);
#11870=AXIS2_PLACEMENT_3D('',#16109,#13138,#13139);
#11871=AXIS2_PLACEMENT_3D('',#16112,#13141,#13142);
#11872=AXIS2_PLACEMENT_3D('',#16113,#13143,#13144);
#11873=AXIS2_PLACEMENT_3D('',#16116,#13146,#13147);
#11874=AXIS2_PLACEMENT_3D('',#16117,#13148,#13149);
#11875=AXIS2_PLACEMENT_3D('',#16119,#13150,#13151);
#11876=AXIS2_PLACEMENT_3D('',#16122,#13153,#13154);
#11877=AXIS2_PLACEMENT_3D('',#16123,#13155,#13156);
#11878=AXIS2_PLACEMENT_3D('',#16124,#13157,#13158);
#11879=AXIS2_PLACEMENT_3D('',#16126,#13159,#13160);
#11880=AXIS2_PLACEMENT_3D('',#16129,#13162,#13163);
#11881=AXIS2_PLACEMENT_3D('',#16130,#13164,#13165);
#11882=AXIS2_PLACEMENT_3D('',#16131,#13166,#13167);
#11883=AXIS2_PLACEMENT_3D('',#16133,#13168,#13169);
#11884=AXIS2_PLACEMENT_3D('',#16136,#13171,#13172);
#11885=AXIS2_PLACEMENT_3D('',#16137,#13173,#13174);
#11886=AXIS2_PLACEMENT_3D('',#16139,#13175,#13176);
#11887=AXIS2_PLACEMENT_3D('',#16140,#13177,#13178);
#11888=AXIS2_PLACEMENT_3D('',#16143,#13180,#13181);
#11889=AXIS2_PLACEMENT_3D('',#16144,#13182,#13183);
#11890=AXIS2_PLACEMENT_3D('',#16146,#13184,#13185);
#11891=AXIS2_PLACEMENT_3D('',#16149,#13187,#13188);
#11892=AXIS2_PLACEMENT_3D('',#16150,#13189,#13190);
#11893=AXIS2_PLACEMENT_3D('',#16152,#13191,#13192);
#11894=AXIS2_PLACEMENT_3D('',#16153,#13193,#13194);
#11895=AXIS2_PLACEMENT_3D('',#16156,#13196,#13197);
#11896=AXIS2_PLACEMENT_3D('',#16157,#13198,#13199);
#11897=AXIS2_PLACEMENT_3D('',#16166,#13204,#13205);
#11898=AXIS2_PLACEMENT_3D('',#16172,#13209,#13210);
#11899=AXIS2_PLACEMENT_3D('',#16178,#13214,#13215);
#11900=AXIS2_PLACEMENT_3D('',#16181,#13218,#13219);
#11901=AXIS2_PLACEMENT_3D('',#16182,#13220,#13221);
#13040=DIRECTION('axis',(0.,0.,1.));
#13041=DIRECTION('refdir',(1.,0.,0.));
#13042=DIRECTION('center_axis',(0.,1.,0.));
#13043=DIRECTION('ref_axis',(1.,0.,0.));
#13044=DIRECTION('center_axis',(0.,1.,0.));
#13045=DIRECTION('ref_axis',(1.,0.,0.));
#13046=DIRECTION('',(0.,1.,0.));
#13047=DIRECTION('center_axis',(0.,-1.,0.));
#13048=DIRECTION('ref_axis',(1.,0.,0.));
#13049=DIRECTION('center_axis',(0.,1.,0.));
#13050=DIRECTION('ref_axis',(1.,0.,0.));
#13051=DIRECTION('center_axis',(0.,1.,0.));
#13052=DIRECTION('ref_axis',(1.,0.,0.));
#13053=DIRECTION('',(0.,1.,0.));
#13054=DIRECTION('center_axis',(0.,-1.,0.));
#13055=DIRECTION('ref_axis',(1.,0.,0.));
#13056=DIRECTION('center_axis',(0.,1.,0.));
#13057=DIRECTION('ref_axis',(1.,0.,0.));
#13058=DIRECTION('center_axis',(0.,1.,0.));
#13059=DIRECTION('ref_axis',(1.,0.,0.));
#13060=DIRECTION('',(0.,1.,0.));
#13061=DIRECTION('center_axis',(0.,-1.,0.));
#13062=DIRECTION('ref_axis',(1.,0.,0.));
#13063=DIRECTION('center_axis',(0.,1.,0.));
#13064=DIRECTION('ref_axis',(1.,0.,0.));
#13065=DIRECTION('center_axis',(0.,1.,0.));
#13066=DIRECTION('ref_axis',(1.,0.,0.));
#13067=DIRECTION('',(0.,1.,0.));
#13068=DIRECTION('center_axis',(0.,-1.,0.));
#13069=DIRECTION('ref_axis',(1.,0.,0.));
#13070=DIRECTION('center_axis',(0.,1.,0.));
#13071=DIRECTION('ref_axis',(1.,0.,0.));
#13072=DIRECTION('center_axis',(0.,1.,0.));
#13073=DIRECTION('ref_axis',(1.,0.,0.));
#13074=DIRECTION('',(0.,1.,0.));
#13075=DIRECTION('center_axis',(0.,-1.,0.));
#13076=DIRECTION('ref_axis',(1.,0.,0.));
#13077=DIRECTION('center_axis',(0.,1.,0.));
#13078=DIRECTION('ref_axis',(1.,0.,0.));
#13079=DIRECTION('center_axis',(0.,1.,0.));
#13080=DIRECTION('ref_axis',(1.,0.,0.));
#13081=DIRECTION('',(0.,1.,0.));
#13082=DIRECTION('center_axis',(0.,-1.,0.));
#13083=DIRECTION('ref_axis',(1.,0.,0.));
#13084=DIRECTION('center_axis',(0.,1.,0.));
#13085=DIRECTION('ref_axis',(1.,0.,0.));
#13086=DIRECTION('center_axis',(0.,1.,0.));
#13087=DIRECTION('ref_axis',(1.,0.,0.));
#13088=DIRECTION('',(0.,1.,0.));
#13089=DIRECTION('center_axis',(0.,1.,0.));
#13090=DIRECTION('ref_axis',(1.,0.,0.));
#13091=DIRECTION('center_axis',(0.,1.,0.));
#13092=DIRECTION('ref_axis',(1.,0.,0.));
#13093=DIRECTION('center_axis',(0.,-1.,0.));
#13094=DIRECTION('ref_axis',(1.,0.,0.));
#13095=DIRECTION('center_axis',(0.,1.,0.));
#13096=DIRECTION('ref_axis',(1.,0.,0.));
#13097=DIRECTION('center_axis',(0.,1.,0.));
#13098=DIRECTION('ref_axis',(1.,0.,0.));
#13099=DIRECTION('',(0.,1.,0.));
#13100=DIRECTION('center_axis',(0.,1.,0.));
#13101=DIRECTION('ref_axis',(1.,0.,0.));
#13102=DIRECTION('center_axis',(0.,1.,0.));
#13103=DIRECTION('ref_axis',(1.,0.,0.));
#13104=DIRECTION('center_axis',(0.,-1.,0.));
#13105=DIRECTION('ref_axis',(1.,0.,0.));
#13106=DIRECTION('center_axis',(0.,1.,0.));
#13107=DIRECTION('ref_axis',(1.,0.,0.));
#13108=DIRECTION('center_axis',(0.,1.,0.));
#13109=DIRECTION('ref_axis',(1.,0.,0.));
#13110=DIRECTION('',(0.,1.,0.));
#13111=DIRECTION('center_axis',(0.,1.,0.));
#13112=DIRECTION('ref_axis',(1.,0.,0.));
#13113=DIRECTION('center_axis',(0.,1.,0.));
#13114=DIRECTION('ref_axis',(1.,0.,0.));
#13115=DIRECTION('center_axis',(0.,-1.,0.));
#13116=DIRECTION('ref_axis',(1.,0.,0.));
#13117=DIRECTION('center_axis',(0.,1.,0.));
#13118=DIRECTION('ref_axis',(1.,0.,0.));
#13119=DIRECTION('center_axis',(0.,1.,0.));
#13120=DIRECTION('ref_axis',(1.,0.,0.));
#13121=DIRECTION('',(0.,1.,0.));
#13122=DIRECTION('center_axis',(0.,1.,0.));
#13123=DIRECTION('ref_axis',(1.,0.,0.));
#13124=DIRECTION('center_axis',(0.,1.,0.));
#13125=DIRECTION('ref_axis',(1.,0.,0.));
#13126=DIRECTION('center_axis',(0.,-1.,0.));
#13127=DIRECTION('ref_axis',(1.,0.,0.));
#13128=DIRECTION('center_axis',(0.,1.,0.));
#13129=DIRECTION('ref_axis',(1.,0.,0.));
#13130=DIRECTION('',(0.,1.,0.));
#13131=DIRECTION('center_axis',(0.,-1.,0.));
#13132=DIRECTION('ref_axis',(1.,0.,0.));
#13133=DIRECTION('center_axis',(0.,1.,0.));
#13134=DIRECTION('ref_axis',(1.,0.,0.));
#13135=DIRECTION('',(0.,1.,0.));
#13136=DIRECTION('center_axis',(0.,-1.,0.));
#13137=DIRECTION('ref_axis',(1.,0.,0.));
#13138=DIRECTION('center_axis',(0.,1.,0.));
#13139=DIRECTION('ref_axis',(1.,0.,0.));
#13140=DIRECTION('',(0.,1.,0.));
#13141=DIRECTION('center_axis',(0.,-1.,0.));
#13142=DIRECTION('ref_axis',(1.,0.,0.));
#13143=DIRECTION('center_axis',(0.,1.,0.));
#13144=DIRECTION('ref_axis',(1.,0.,0.));
#13145=DIRECTION('',(0.,1.,0.));
#13146=DIRECTION('center_axis',(0.,-1.,0.));
#13147=DIRECTION('ref_axis',(1.,0.,0.));
#13148=DIRECTION('center_axis',(0.,0.,1.));
#13149=DIRECTION('ref_axis',(1.,0.,0.));
#13150=DIRECTION('center_axis',(0.,0.,1.));
#13151=DIRECTION('ref_axis',(1.,0.,0.));
#13152=DIRECTION('',(0.,0.,1.));
#13153=DIRECTION('center_axis',(0.,0.,1.));
#13154=DIRECTION('ref_axis',(1.,0.,0.));
#13155=DIRECTION('center_axis',(0.,0.,1.));
#13156=DIRECTION('ref_axis',(1.,0.,0.));
#13157=DIRECTION('center_axis',(0.,0.,1.));
#13158=DIRECTION('ref_axis',(1.,0.,0.));
#13159=DIRECTION('center_axis',(0.,0.,1.));
#13160=DIRECTION('ref_axis',(1.,0.,0.));
#13161=DIRECTION('',(0.,0.,1.));
#13162=DIRECTION('center_axis',(0.,0.,1.));
#13163=DIRECTION('ref_axis',(1.,0.,0.));
#13164=DIRECTION('center_axis',(0.,0.,1.));
#13165=DIRECTION('ref_axis',(1.,0.,0.));
#13166=DIRECTION('center_axis',(0.,1.,0.));
#13167=DIRECTION('ref_axis',(1.,0.,0.));
#13168=DIRECTION('center_axis',(0.,1.,0.));
#13169=DIRECTION('ref_axis',(1.,0.,0.));
#13170=DIRECTION('',(0.,1.,0.));
#13171=DIRECTION('center_axis',(0.,1.,0.));
#13172=DIRECTION('ref_axis',(1.,0.,0.));
#13173=DIRECTION('center_axis',(0.,1.,0.));
#13174=DIRECTION('ref_axis',(1.,0.,0.));
#13175=DIRECTION('center_axis',(0.,-1.,0.));
#13176=DIRECTION('ref_axis',(1.,0.,0.));
#13177=DIRECTION('center_axis',(0.,1.,0.));
#13178=DIRECTION('ref_axis',(1.,0.,0.));
#13179=DIRECTION('',(0.,1.,0.));
#13180=DIRECTION('center_axis',(0.,-1.,0.));
#13181=DIRECTION('ref_axis',(1.,0.,0.));
#13182=DIRECTION('center_axis',(0.,1.,0.));
#13183=DIRECTION('ref_axis',(1.,0.,0.));
#13184=DIRECTION('center_axis',(0.,1.,0.));
#13185=DIRECTION('ref_axis',(1.,0.,0.));
#13186=DIRECTION('',(0.,1.,0.));
#13187=DIRECTION('center_axis',(0.,1.,0.));
#13188=DIRECTION('ref_axis',(1.,0.,0.));
#13189=DIRECTION('center_axis',(0.,1.,0.));
#13190=DIRECTION('ref_axis',(1.,0.,0.));
#13191=DIRECTION('center_axis',(0.,-1.,0.));
#13192=DIRECTION('ref_axis',(1.,0.,0.));
#13193=DIRECTION('center_axis',(0.,1.,0.));
#13194=DIRECTION('ref_axis',(1.,0.,0.));
#13195=DIRECTION('',(0.,1.,0.));
#13196=DIRECTION('center_axis',(0.,-1.,0.));
#13197=DIRECTION('ref_axis',(1.,0.,0.));
#13198=DIRECTION('center_axis',(0.,1.,0.));
#13199=DIRECTION('ref_axis',(-1.,0.,0.));
#13200=DIRECTION('',(-1.,0.,0.));
#13201=DIRECTION('',(0.,0.,1.));
#13202=DIRECTION('',(-1.,0.,0.));
#13203=DIRECTION('',(0.,0.,1.));
#13204=DIRECTION('center_axis',(1.,0.,0.));
#13205=DIRECTION('ref_axis',(0.,1.,0.));
#13206=DIRECTION('',(0.,1.,0.));
#13207=DIRECTION('',(0.,1.,0.));
#13208=DIRECTION('',(0.,0.,1.));
#13209=DIRECTION('center_axis',(0.,-1.,0.));
#13210=DIRECTION('ref_axis',(1.,0.,0.));
#13211=DIRECTION('',(1.,0.,0.));
#13212=DIRECTION('',(1.,0.,0.));
#13213=DIRECTION('',(0.,0.,1.));
#13214=DIRECTION('center_axis',(-1.,0.,0.));
#13215=DIRECTION('ref_axis',(0.,-1.,0.));
#13216=DIRECTION('',(0.,-1.,0.));
#13217=DIRECTION('',(0.,-1.,0.));
#13218=DIRECTION('center_axis',(0.,0.,1.));
#13219=DIRECTION('ref_axis',(1.,0.,0.));
#13220=DIRECTION('center_axis',(0.,0.,1.));
#13221=DIRECTION('ref_axis',(1.,0.,0.));
#16028=CARTESIAN_POINT('',(0.,0.,0.));
#16029=CARTESIAN_POINT('Origin',(6.,-4.5,7.6));
#16030=CARTESIAN_POINT('',(5.835,-4.4,7.6));
#16031=CARTESIAN_POINT('Origin',(6.,-4.4,7.6));
#16032=CARTESIAN_POINT('',(5.835,-2.6,7.6));
#16033=CARTESIAN_POINT('',(5.835,-4.5,7.6));
#16034=CARTESIAN_POINT('Origin',(6.,-2.6,7.6));
#16035=CARTESIAN_POINT('Origin',(3.74833395016046,-4.5,3.7));
#16036=CARTESIAN_POINT('',(3.58333395016046,-4.4,3.7));
#16037=CARTESIAN_POINT('Origin',(3.74833395016046,-4.4,3.7));
#16038=CARTESIAN_POINT('',(3.58333395016046,-2.6,3.7));
#16039=CARTESIAN_POINT('',(3.58333395016046,-4.5,3.7));
#16040=CARTESIAN_POINT('Origin',(3.74833395016046,-2.6,3.7));
#16041=CARTESIAN_POINT('Origin',(8.25166604983954,-4.5,3.7));
#16042=CARTESIAN_POINT('',(8.08666604983954,-4.4,3.7));
#16043=CARTESIAN_POINT('Origin',(8.25166604983954,-4.4,3.7));
#16044=CARTESIAN_POINT('',(8.08666604983954,-2.6,3.7));
#16045=CARTESIAN_POINT('',(8.08666604983954,-4.5,3.7));
#16046=CARTESIAN_POINT('Origin',(8.25166604983954,-2.6,3.7));
#16047=CARTESIAN_POINT('Origin',(1.16341445918999E-16,-4.5,6.9));
#16048=CARTESIAN_POINT('',(-0.165,-4.4,6.9));
#16049=CARTESIAN_POINT('Origin',(1.16341445918999E-16,-4.4,6.9));
#16050=CARTESIAN_POINT('',(-0.165,-2.6,6.9));
#16051=CARTESIAN_POINT('',(-0.165,-4.5,6.9));
#16052=CARTESIAN_POINT('Origin',(1.16341445918999E-16,-2.6,6.9));
#16053=CARTESIAN_POINT('Origin',(-1.64544826719043,-4.5,4.05));
#16054=CARTESIAN_POINT('',(-1.81044826719043,-4.4,4.05));
#16055=CARTESIAN_POINT('Origin',(-1.64544826719043,-4.4,4.05));
#16056=CARTESIAN_POINT('',(-1.81044826719043,-2.6,4.05));
#16057=CARTESIAN_POINT('',(-1.81044826719043,-4.5,4.05));
#16058=CARTESIAN_POINT('Origin',(-1.64544826719043,-2.6,4.05));
#16059=CARTESIAN_POINT('Origin',(1.64544826719043,-4.5,4.05));
#16060=CARTESIAN_POINT('',(1.48044826719043,-4.4,4.05));
#16061=CARTESIAN_POINT('Origin',(1.64544826719043,-4.4,4.05));
#16062=CARTESIAN_POINT('',(1.48044826719043,-2.6,4.05));
#16063=CARTESIAN_POINT('',(1.48044826719043,-4.5,4.05));
#16064=CARTESIAN_POINT('Origin',(1.64544826719043,-2.6,4.05));
#16065=CARTESIAN_POINT('Origin',(10.,-4.5,2.));
#16066=CARTESIAN_POINT('',(9.525,-4.4,2.));
#16067=CARTESIAN_POINT('Origin',(10.,-4.4,2.));
#16068=CARTESIAN_POINT('',(9.525,-3.9,2.));
#16069=CARTESIAN_POINT('',(9.525,-4.5,2.));
#16070=CARTESIAN_POINT('Origin',(10.,-3.9,2.));
#16071=CARTESIAN_POINT('Origin',(10.,-3.9,2.));
#16072=CARTESIAN_POINT('',(9.725,-3.9,2.));
#16073=CARTESIAN_POINT('Origin',(10.,-3.9,2.));
#16074=CARTESIAN_POINT('Origin',(-2.,-4.5,9.));
#16075=CARTESIAN_POINT('',(-2.475,-4.4,9.));
#16076=CARTESIAN_POINT('Origin',(-2.,-4.4,9.));
#16077=CARTESIAN_POINT('',(-2.475,-3.9,9.));
#16078=CARTESIAN_POINT('',(-2.475,-4.5,9.));
#16079=CARTESIAN_POINT('Origin',(-2.,-3.9,9.));
#16080=CARTESIAN_POINT('Origin',(-2.,-3.9,9.));
#16081=CARTESIAN_POINT('',(-2.275,-3.9,9.));
#16082=CARTESIAN_POINT('Origin',(-2.,-3.9,9.));
#16083=CARTESIAN_POINT('Origin',(-2.,-4.5,2.));
#16084=CARTESIAN_POINT('',(-2.475,-4.4,2.));
#16085=CARTESIAN_POINT('Origin',(-2.,-4.4,2.));
#16086=CARTESIAN_POINT('',(-2.475,-3.9,2.));
#16087=CARTESIAN_POINT('',(-2.475,-4.5,2.));
#16088=CARTESIAN_POINT('Origin',(-2.,-3.9,2.));
#16089=CARTESIAN_POINT('Origin',(-2.,-3.9,2.));
#16090=CARTESIAN_POINT('',(-2.275,-3.9,2.));
#16091=CARTESIAN_POINT('Origin',(-2.,-3.9,2.));
#16092=CARTESIAN_POINT('Origin',(10.,-4.5,9.));
#16093=CARTESIAN_POINT('',(9.525,-4.4,9.));
#16094=CARTESIAN_POINT('Origin',(10.,-4.4,9.));
#16095=CARTESIAN_POINT('',(9.525,-3.9,9.));
#16096=CARTESIAN_POINT('',(9.525,-4.5,9.));
#16097=CARTESIAN_POINT('Origin',(10.,-3.9,9.));
#16098=CARTESIAN_POINT('Origin',(10.,-3.9,9.));
#16099=CARTESIAN_POINT('',(9.725,-3.9,9.));
#16100=CARTESIAN_POINT('Origin',(10.,-3.9,9.));
#16101=CARTESIAN_POINT('Origin',(10.,-4.5,2.));
#16102=CARTESIAN_POINT('',(9.725,-2.6,2.));
#16103=CARTESIAN_POINT('',(9.725,-4.5,2.));
#16104=CARTESIAN_POINT('Origin',(10.,-2.6,2.));
#16105=CARTESIAN_POINT('Origin',(-2.,-4.5,9.));
#16106=CARTESIAN_POINT('',(-2.275,-2.6,9.));
#16107=CARTESIAN_POINT('',(-2.275,-4.5,9.));
#16108=CARTESIAN_POINT('Origin',(-2.,-2.6,9.));
#16109=CARTESIAN_POINT('Origin',(-2.,-4.5,2.));
#16110=CARTESIAN_POINT('',(-2.275,-2.6,2.));
#16111=CARTESIAN_POINT('',(-2.275,-4.5,2.));
#16112=CARTESIAN_POINT('Origin',(-2.,-2.6,2.));
#16113=CARTESIAN_POINT('Origin',(10.,-4.5,9.));
#16114=CARTESIAN_POINT('',(9.725,-2.6,9.));
#16115=CARTESIAN_POINT('',(9.725,-4.5,9.));
#16116=CARTESIAN_POINT('Origin',(10.,-2.6,9.));
#16117=CARTESIAN_POINT('Origin',(10.,-3.5,-0.1));
#16118=CARTESIAN_POINT('',(9.75,-3.5,0.));
#16119=CARTESIAN_POINT('Origin',(10.,-3.5,0.));
#16120=CARTESIAN_POINT('',(9.75,-3.5,1.7));
#16121=CARTESIAN_POINT('',(9.75,-3.5,-0.1));
#16122=CARTESIAN_POINT('Origin',(10.,-3.5,1.7));
#16123=CARTESIAN_POINT('Origin',(10.,-3.5,1.7));
#16124=CARTESIAN_POINT('Origin',(-2.,-3.5,-0.1));
#16125=CARTESIAN_POINT('',(-2.25,-3.5,0.));
#16126=CARTESIAN_POINT('Origin',(-2.,-3.5,0.));
#16127=CARTESIAN_POINT('',(-2.25,-3.5,1.7));
#16128=CARTESIAN_POINT('',(-2.25,-3.5,-0.1));
#16129=CARTESIAN_POINT('Origin',(-2.,-3.5,1.7));
#16130=CARTESIAN_POINT('Origin',(-2.,-3.5,1.7));
#16131=CARTESIAN_POINT('Origin',(6.,-4.5,5.));
#16132=CARTESIAN_POINT('',(3.65,-4.4,5.));
#16133=CARTESIAN_POINT('Origin',(6.,-4.4,5.));
#16134=CARTESIAN_POINT('',(3.65,-2.8,5.));
#16135=CARTESIAN_POINT('',(3.65,-4.5,5.));
#16136=CARTESIAN_POINT('Origin',(6.,-2.8,5.));
#16137=CARTESIAN_POINT('Origin',(6.,-2.8,5.));
#16138=CARTESIAN_POINT('',(3.85,-2.8,5.));
#16139=CARTESIAN_POINT('Origin',(6.,-2.8,5.));
#16140=CARTESIAN_POINT('Origin',(6.,-4.5,5.));
#16141=CARTESIAN_POINT('',(3.85,-2.6,5.));
#16142=CARTESIAN_POINT('',(3.85,-4.5,5.));
#16143=CARTESIAN_POINT('Origin',(6.,-2.6,5.));
#16144=CARTESIAN_POINT('Origin',(0.,-4.5,5.));
#16145=CARTESIAN_POINT('',(-1.6,-4.4,5.));
#16146=CARTESIAN_POINT('Origin',(0.,-4.4,5.));
#16147=CARTESIAN_POINT('',(-1.6,-3.,5.));
#16148=CARTESIAN_POINT('',(-1.6,-4.5,5.));
#16149=CARTESIAN_POINT('Origin',(0.,-3.,5.));
#16150=CARTESIAN_POINT('Origin',(0.,-3.,5.));
#16151=CARTESIAN_POINT('',(-1.4,-3.,5.));
#16152=CARTESIAN_POINT('Origin',(0.,-3.,5.));
#16153=CARTESIAN_POINT('Origin',(0.,-4.5,5.));
#16154=CARTESIAN_POINT('',(-1.4,-2.6,5.));
#16155=CARTESIAN_POINT('',(-1.4,-4.5,5.));
#16156=CARTESIAN_POINT('Origin',(0.,-2.6,5.));
#16157=CARTESIAN_POINT('Origin',(11.,-2.6,0.));
#16158=CARTESIAN_POINT('',(11.,-2.6,0.));
#16159=CARTESIAN_POINT('',(-3.,-2.6,0.));
#16160=CARTESIAN_POINT('',(11.,-2.6,0.));
#16161=CARTESIAN_POINT('',(-3.,-2.6,10.));
#16162=CARTESIAN_POINT('',(-3.,-2.6,0.));
#16163=CARTESIAN_POINT('',(11.,-2.6,10.));
#16164=CARTESIAN_POINT('',(11.,-2.6,10.));
#16165=CARTESIAN_POINT('',(11.,-2.6,0.));
#16166=CARTESIAN_POINT('Origin',(11.,-4.4,0.));
#16167=CARTESIAN_POINT('',(11.,-4.4,0.));
#16168=CARTESIAN_POINT('',(11.,-4.4,0.));
#16169=CARTESIAN_POINT('',(11.,-4.4,10.));
#16170=CARTESIAN_POINT('',(11.,-4.4,10.));
#16171=CARTESIAN_POINT('',(11.,-4.4,0.));
#16172=CARTESIAN_POINT('Origin',(-3.,-4.4,0.));
#16173=CARTESIAN_POINT('',(-3.,-4.4,0.));
#16174=CARTESIAN_POINT('',(-3.,-4.4,0.));
#16175=CARTESIAN_POINT('',(-3.,-4.4,10.));
#16176=CARTESIAN_POINT('',(-3.,-4.4,10.));
#16177=CARTESIAN_POINT('',(-3.,-4.4,0.));
#16178=CARTESIAN_POINT('Origin',(-3.,-2.6,0.));
#16179=CARTESIAN_POINT('',(-3.,-2.6,0.));
#16180=CARTESIAN_POINT('',(-3.,-2.6,10.));
#16181=CARTESIAN_POINT('Origin',(4.,-3.5,10.));
#16182=CARTESIAN_POINT('Origin',(4.,-3.5,0.));
#53813=UNCERTAINTY_MEASURE_WITH_UNIT(LENGTH_MEASURE(0.001),#53910,
'DISTANCE_ACCURACY_VALUE',
'Maximum model space distance between geometric entities at asserted c
onnectivities');
#53859=UNCERTAINTY_MEASURE_WITH_UNIT(LENGTH_MEASURE(0.001),#53910,
'DISTANCE_ACCURACY_VALUE',
'Maximum model space distance between geometric entities at asserted c
onnectivities');
#53863=(
GEOMETRIC_REPRESENTATION_CONTEXT(3)
GLOBAL_UNCERTAINTY_ASSIGNED_CONTEXT((#53813))
GLOBAL_UNIT_ASSIGNED_CONTEXT((#53910,#53912,#53913))
REPRESENTATION_CONTEXT('','3D')
);
#53909=(
GEOMETRIC_REPRESENTATION_CONTEXT(3)
GLOBAL_UNCERTAINTY_ASSIGNED_CONTEXT((#53859))
GLOBAL_UNIT_ASSIGNED_CONTEXT((#53910,#53912,#53913))
REPRESENTATION_CONTEXT('','3D')
);
#53910=(
LENGTH_UNIT()
NAMED_UNIT(*)
SI_UNIT(.CENTI.,.METRE.)
);
#53912=(
NAMED_UNIT(*)
PLANE_ANGLE_UNIT()
SI_UNIT($,.RADIAN.)
);
#53913=(
NAMED_UNIT(*)
SI_UNIT($,.STERADIAN.)
SOLID_ANGLE_UNIT()
);
#53917=SHAPE_DEFINITION_REPRESENTATION(#53966,#54089);
#53966=PRODUCT_DEFINITION_SHAPE('',$,#54139);
#54089=SHAPE_REPRESENTATION('',(#11827),#53863);
#54135=PRODUCT_DEFINITION_CONTEXT('part definition',#54284,'design');
#54139=PRODUCT_DEFINITION('Front plate','Front plate',#54188,#54135);
#54188=PRODUCT_DEFINITION_FORMATION('',$,#54289);
#54284=APPLICATION_CONTEXT(
'Core Data for Automotive Mechanical Design Process');
#54285=PRODUCT_CONTEXT('part definition',#54284,'mechanical');
#54289=PRODUCT('Front plate','Front plate','Front plate',(#54285));
#54405=COLOUR_RGB('Off White',0.89,0.88,0.83);
#54406=FILL_AREA_STYLE_COLOUR('',#54405);
#54407=FILL_AREA_STYLE('',(#54406));
#54408=SURFACE_STYLE_FILL_AREA(#54407);
#54409=SURFACE_SIDE_STYLE('',(#54408));
#54410=SURFACE_STYLE_USAGE(.BOTH.,#54409);
#54411=PRESENTATION_STYLE_ASSIGNMENT((#54410));
ENDSEC;
END-ISO-10303-21;
